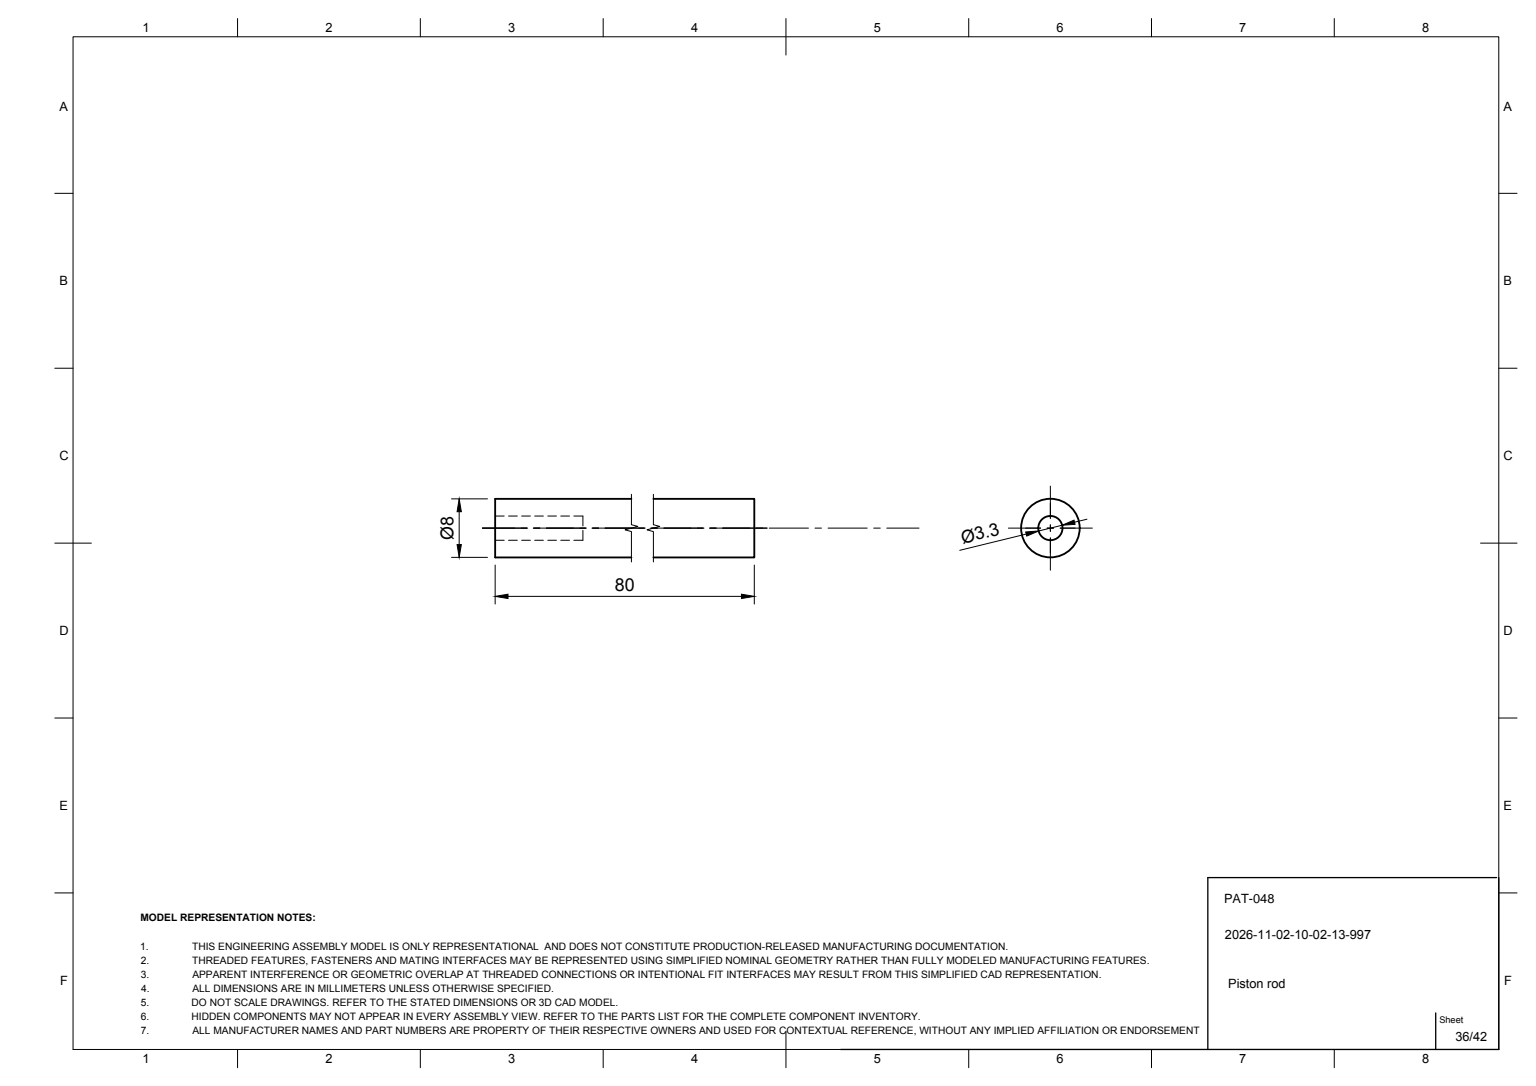
ISO-10303-21;
HEADER;
/* Generated by software containing ST-Developer
 * from STEP Tools, Inc. (www.steptools.com) 
 */

FILE_DESCRIPTION(
/* description */ ('Guided pneumatic stop gate'),
/* implementation_level */ '2;1');

FILE_NAME(
/* name */ 'Piston rod.step',
/* time_stamp */ '2026-10-27T21:43:45-07:00',
/* author */ (''),
/* organization */ (''),
/* preprocessor_version */ 'ST-DEVELOPER v20.2',
/* originating_system */ 'Autodesk Translation Framework v15.17.0.0',
/* authorisation */ '');

FILE_SCHEMA (('AUTOMOTIVE_DESIGN { 1 0 10303 214 3 1 1 }'));
ENDSEC;

DATA;
#10=MECHANICAL_DESIGN_GEOMETRIC_PRESENTATION_REPRESENTATION('',(#565),#14392);
#481=SHAPE_REPRESENTATION_RELATIONSHIP('SRR','None',#14618,#523);
#523=ADVANCED_BREP_SHAPE_REPRESENTATION('',(#604),#14380);
#565=STYLED_ITEM('',(#14891),#604);
#604=MANIFOLD_SOLID_BREP('Body1',#7908);
#796=FACE_BOUND('',#2147,.T.);
#1048=PLANE('',#9184);
#1049=PLANE('',#9188);
#1050=PLANE('',#9189);
#1487=FACE_OUTER_BOUND('',#2143,.T.);
#1488=FACE_OUTER_BOUND('',#2144,.T.);
#1489=FACE_OUTER_BOUND('',#2145,.T.);
#1490=FACE_OUTER_BOUND('',#2146,.T.);
#1491=FACE_OUTER_BOUND('',#2148,.T.);
#2143=EDGE_LOOP('',(#6806,#6807,#6808,#6809));
#2144=EDGE_LOOP('',(#6810));
#2145=EDGE_LOOP('',(#6811,#6812,#6813,#6814));
#2146=EDGE_LOOP('',(#6815));
#2147=EDGE_LOOP('',(#6816));
#2148=EDGE_LOOP('',(#6817));
#2691=LINE('',#13649,#3236);
#2692=LINE('',#13656,#3237);
#3236=VECTOR('',#11392,0.165);
#3237=VECTOR('',#11401,0.4);
#3674=CIRCLE('',#9182,0.165);
#3675=CIRCLE('',#9183,0.165);
#3676=CIRCLE('',#9186,0.4);
#3677=CIRCLE('',#9187,0.4);
#4216=VERTEX_POINT('',#13646);
#4217=VERTEX_POINT('',#13648);
#4218=VERTEX_POINT('',#13653);
#4219=VERTEX_POINT('',#13655);
#5101=EDGE_CURVE('',#4216,#4216,#3674,.T.);
#5102=EDGE_CURVE('',#4216,#4217,#2691,.T.);
#5103=EDGE_CURVE('',#4217,#4217,#3675,.T.);
#5104=EDGE_CURVE('',#4218,#4218,#3676,.T.);
#5105=EDGE_CURVE('',#4218,#4219,#2692,.T.);
#5106=EDGE_CURVE('',#4219,#4219,#3677,.T.);
#6806=ORIENTED_EDGE('',*,*,#5101,.F.);
#6807=ORIENTED_EDGE('',*,*,#5102,.T.);
#6808=ORIENTED_EDGE('',*,*,#5103,.F.);
#6809=ORIENTED_EDGE('',*,*,#5102,.F.);
#6810=ORIENTED_EDGE('',*,*,#5101,.T.);
#6811=ORIENTED_EDGE('',*,*,#5104,.F.);
#6812=ORIENTED_EDGE('',*,*,#5105,.T.);
#6813=ORIENTED_EDGE('',*,*,#5106,.T.);
#6814=ORIENTED_EDGE('',*,*,#5105,.F.);
#6815=ORIENTED_EDGE('',*,*,#5104,.T.);
#6816=ORIENTED_EDGE('',*,*,#5103,.T.);
#6817=ORIENTED_EDGE('',*,*,#5106,.F.);
#7375=CYLINDRICAL_SURFACE('',#9181,0.165);
#7376=CYLINDRICAL_SURFACE('',#9185,0.4);
#7769=ADVANCED_FACE('',(#1487),#7375,.F.);
#7770=ADVANCED_FACE('',(#1488),#1048,.T.);
#7771=ADVANCED_FACE('',(#1489),#7376,.T.);
#7772=ADVANCED_FACE('',(#1490,#796),#1049,.T.);
#7773=ADVANCED_FACE('',(#1491),#1050,.F.);
#7908=CLOSED_SHELL('',(#7769,#7770,#7771,#7772,#7773));
#9180=AXIS2_PLACEMENT_3D('',#13644,#11386,#11387);
#9181=AXIS2_PLACEMENT_3D('',#13645,#11388,#11389);
#9182=AXIS2_PLACEMENT_3D('',#13647,#11390,#11391);
#9183=AXIS2_PLACEMENT_3D('',#13650,#11393,#11394);
#9184=AXIS2_PLACEMENT_3D('',#13651,#11395,#11396);
#9185=AXIS2_PLACEMENT_3D('',#13652,#11397,#11398);
#9186=AXIS2_PLACEMENT_3D('',#13654,#11399,#11400);
#9187=AXIS2_PLACEMENT_3D('',#13657,#11402,#11403);
#9188=AXIS2_PLACEMENT_3D('',#13658,#11404,#11405);
#9189=AXIS2_PLACEMENT_3D('',#13659,#11406,#11407);
#11386=DIRECTION('axis',(0.,0.,1.));
#11387=DIRECTION('refdir',(1.,0.,0.));
#11388=DIRECTION('center_axis',(0.,1.,0.));
#11389=DIRECTION('ref_axis',(1.,0.,0.));
#11390=DIRECTION('center_axis',(0.,1.,0.));
#11391=DIRECTION('ref_axis',(1.,0.,0.));
#11392=DIRECTION('',(0.,1.,0.));
#11393=DIRECTION('center_axis',(0.,-1.,0.));
#11394=DIRECTION('ref_axis',(1.,0.,0.));
#11395=DIRECTION('center_axis',(0.,1.,0.));
#11396=DIRECTION('ref_axis',(1.,0.,0.));
#11397=DIRECTION('center_axis',(0.,1.,0.));
#11398=DIRECTION('ref_axis',(1.,0.,0.));
#11399=DIRECTION('center_axis',(0.,1.,0.));
#11400=DIRECTION('ref_axis',(1.,0.,0.));
#11401=DIRECTION('',(0.,-1.,0.));
#11402=DIRECTION('center_axis',(0.,1.,0.));
#11403=DIRECTION('ref_axis',(1.,0.,0.));
#11404=DIRECTION('center_axis',(0.,1.,0.));
#11405=DIRECTION('ref_axis',(1.,0.,0.));
#11406=DIRECTION('center_axis',(0.,1.,0.));
#11407=DIRECTION('ref_axis',(1.,0.,0.));
#13644=CARTESIAN_POINT('',(0.,0.,0.));
#13645=CARTESIAN_POINT('Origin',(0.,1.2,4.5));
#13646=CARTESIAN_POINT('',(-0.165,1.2,4.5));
#13647=CARTESIAN_POINT('Origin',(0.,1.2,4.5));
#13648=CARTESIAN_POINT('',(-0.165,2.4,4.5));
#13649=CARTESIAN_POINT('',(-0.165,1.2,4.5));
#13650=CARTESIAN_POINT('Origin',(0.,2.4,4.5));
#13651=CARTESIAN_POINT('Origin',(0.,1.2,4.5));
#13652=CARTESIAN_POINT('Origin',(0.,-5.6,4.5));
#13653=CARTESIAN_POINT('',(-0.4,2.4,4.5));
#13654=CARTESIAN_POINT('Origin',(0.,2.4,4.5));
#13655=CARTESIAN_POINT('',(-0.4,-5.6,4.5));
#13656=CARTESIAN_POINT('',(-0.4,-5.6,4.5));
#13657=CARTESIAN_POINT('Origin',(0.,-5.6,4.5));
#13658=CARTESIAN_POINT('Origin',(0.,2.4,4.5));
#13659=CARTESIAN_POINT('Origin',(0.,-5.6,4.5));
#14332=UNCERTAINTY_MEASURE_WITH_UNIT(LENGTH_MEASURE(0.001),#14393,
'DISTANCE_ACCURACY_VALUE',
'Maximum model space distance between geometric entities at asserted c
onnectivities');
#14344=UNCERTAINTY_MEASURE_WITH_UNIT(LENGTH_MEASURE(0.001),#14393,
'DISTANCE_ACCURACY_VALUE',
'Maximum model space distance between geometric entities at asserted c
onnectivities');
#14380=(
GEOMETRIC_REPRESENTATION_CONTEXT(3)
GLOBAL_UNCERTAINTY_ASSIGNED_CONTEXT((#14332))
GLOBAL_UNIT_ASSIGNED_CONTEXT((#14393,#14395,#14396))
REPRESENTATION_CONTEXT('','3D')
);
#14392=(
GEOMETRIC_REPRESENTATION_CONTEXT(3)
GLOBAL_UNCERTAINTY_ASSIGNED_CONTEXT((#14344))
GLOBAL_UNIT_ASSIGNED_CONTEXT((#14393,#14395,#14396))
REPRESENTATION_CONTEXT('','3D')
);
#14393=(
LENGTH_UNIT()
NAMED_UNIT(*)
SI_UNIT(.CENTI.,.METRE.)
);
#14395=(
NAMED_UNIT(*)
PLANE_ANGLE_UNIT()
SI_UNIT($,.RADIAN.)
);
#14396=(
NAMED_UNIT(*)
SI_UNIT($,.STERADIAN.)
SOLID_ANGLE_UNIT()
);
#14432=SHAPE_DEFINITION_REPRESENTATION(#14551,#14618);
#14551=PRODUCT_DEFINITION_SHAPE('',$,#14666);
#14618=SHAPE_REPRESENTATION('',(#9180),#14380);
#14630=PRODUCT_DEFINITION_CONTEXT('part definition',#14773,'design');
#14666=PRODUCT_DEFINITION('Piston rod','Piston rod',#14713,#14630);
#14713=PRODUCT_DEFINITION_FORMATION('',$,#14810);
#14773=APPLICATION_CONTEXT(
'Core Data for Automotive Mechanical Design Process');
#14774=PRODUCT_CONTEXT('part definition',#14773,'mechanical');
#14810=PRODUCT('Piston rod','Piston rod','Piston rod',(#14774));
#14885=COLOUR_RGB('Grey',0.48,0.52,0.57);
#14886=FILL_AREA_STYLE_COLOUR('',#14885);
#14887=FILL_AREA_STYLE('',(#14886));
#14888=SURFACE_STYLE_FILL_AREA(#14887);
#14889=SURFACE_SIDE_STYLE('',(#14888));
#14890=SURFACE_STYLE_USAGE(.BOTH.,#14889);
#14891=PRESENTATION_STYLE_ASSIGNMENT((#14890));
ENDSEC;
END-ISO-10303-21;
